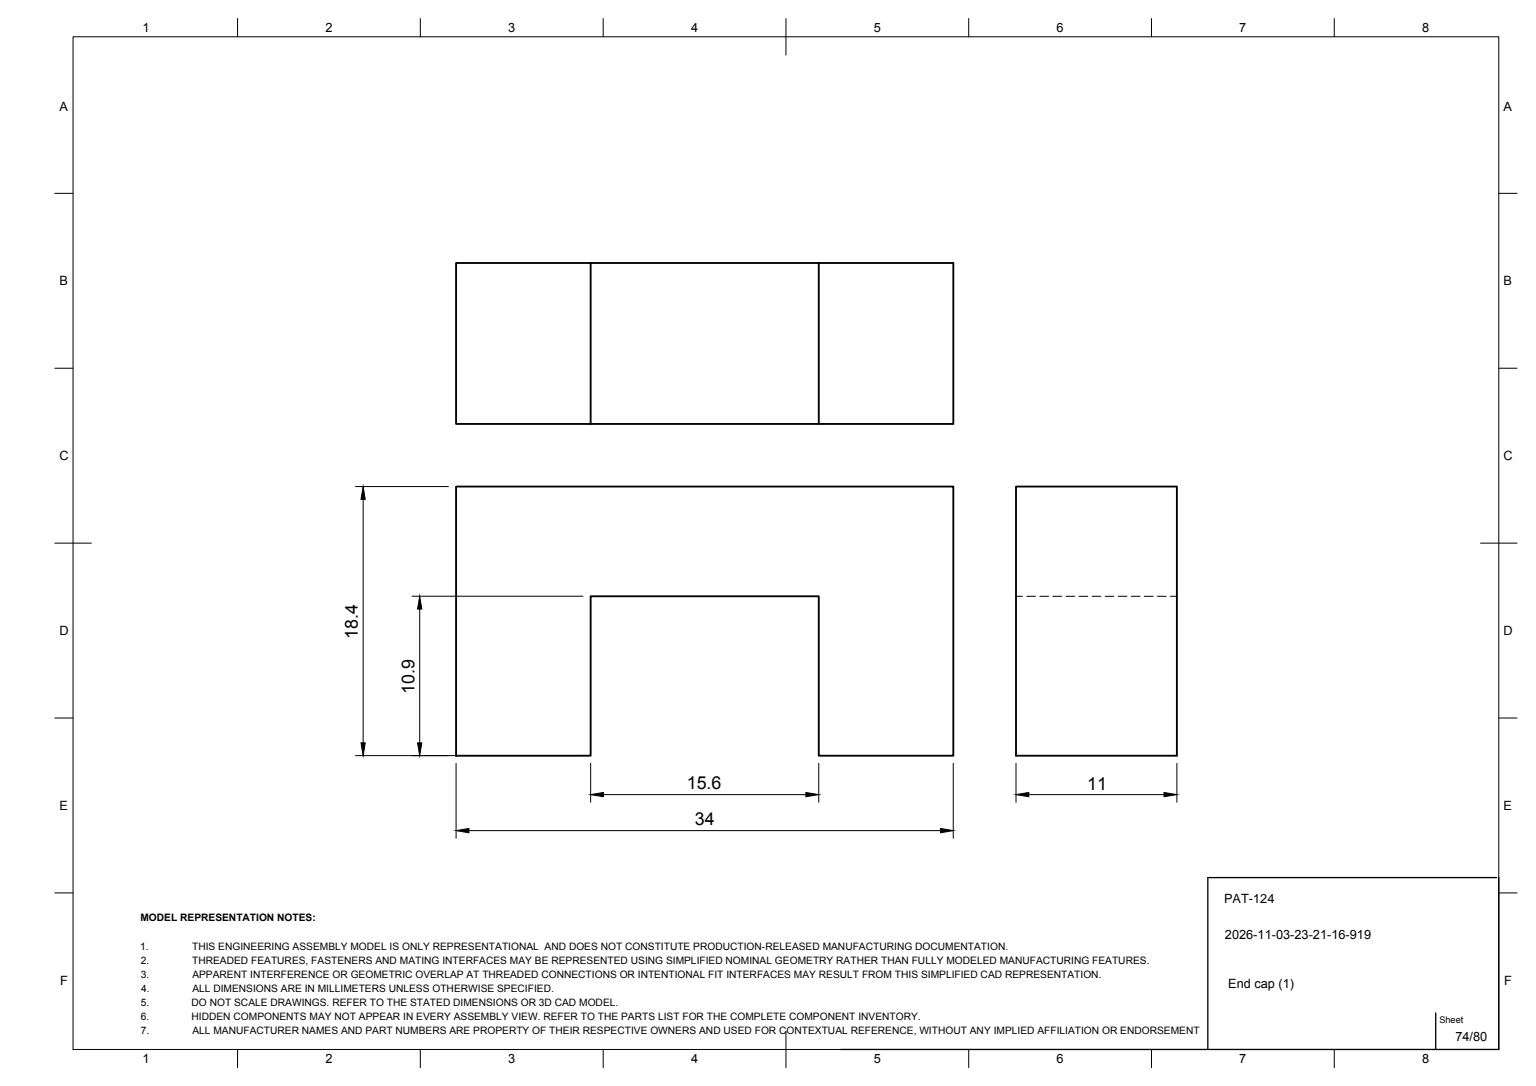
ISO-10303-21;
HEADER;
/* Generated by software containing ST-Developer
 * from STEP Tools, Inc. (www.steptools.com) 
 */

FILE_DESCRIPTION(
/* description */ ('XY cross-slide table'),
/* implementation_level */ '2;1');

FILE_NAME(
/* name */ 'End cap (1).step',
/* time_stamp */ '2026-10-28T03:22:46-07:00',
/* author */ (''),
/* organization */ (''),
/* preprocessor_version */ 'ST-DEVELOPER v20.2',
/* originating_system */ 'Autodesk Translation Framework v15.17.0.0',
/* authorisation */ '');

FILE_SCHEMA (('AUTOMOTIVE_DESIGN { 1 0 10303 214 3 1 1 }'));
ENDSEC;

DATA;
#10=MECHANICAL_DESIGN_GEOMETRIC_PRESENTATION_REPRESENTATION('',(#1767),#62984);
#1571=SHAPE_REPRESENTATION_RELATIONSHIP('SRR','None',#63430,#1654);
#1654=ADVANCED_BREP_SHAPE_REPRESENTATION('',(#1875),#62967);
#1767=STYLED_ITEM('',(#63926),#1875);
#1875=MANIFOLD_SOLID_BREP('Body1',#23066);
#2759=PLANE('',#25957);
#2760=PLANE('',#25958);
#2761=PLANE('',#25959);
#2762=PLANE('',#25960);
#2763=PLANE('',#25961);
#2764=PLANE('',#25962);
#2765=PLANE('',#25963);
#2766=PLANE('',#25964);
#2767=PLANE('',#25965);
#2768=PLANE('',#25966);
#3867=FACE_OUTER_BOUND('',#5551,.T.);
#3868=FACE_OUTER_BOUND('',#5552,.T.);
#3869=FACE_OUTER_BOUND('',#5553,.T.);
#3870=FACE_OUTER_BOUND('',#5554,.T.);
#3871=FACE_OUTER_BOUND('',#5555,.T.);
#3872=FACE_OUTER_BOUND('',#5556,.T.);
#3873=FACE_OUTER_BOUND('',#5557,.T.);
#3874=FACE_OUTER_BOUND('',#5558,.T.);
#3875=FACE_OUTER_BOUND('',#5559,.T.);
#3876=FACE_OUTER_BOUND('',#5560,.T.);
#5551=EDGE_LOOP('',(#19482,#19483,#19484,#19485));
#5552=EDGE_LOOP('',(#19486,#19487,#19488,#19489));
#5553=EDGE_LOOP('',(#19490,#19491,#19492,#19493));
#5554=EDGE_LOOP('',(#19494,#19495,#19496,#19497));
#5555=EDGE_LOOP('',(#19498,#19499,#19500,#19501));
#5556=EDGE_LOOP('',(#19502,#19503,#19504,#19505));
#5557=EDGE_LOOP('',(#19506,#19507,#19508,#19509));
#5558=EDGE_LOOP('',(#19510,#19511,#19512,#19513));
#5559=EDGE_LOOP('',(#19514,#19515,#19516,#19517,#19518,#19519,#19520,#19521));
#5560=EDGE_LOOP('',(#19522,#19523,#19524,#19525,#19526,#19527,#19528,#19529));
#7028=LINE('',#50118,#8515);
#7029=LINE('',#50120,#8516);
#7030=LINE('',#50122,#8517);
#7031=LINE('',#50123,#8518);
#7032=LINE('',#50126,#8519);
#7033=LINE('',#50128,#8520);
#7034=LINE('',#50129,#8521);
#7035=LINE('',#50132,#8522);
#7036=LINE('',#50134,#8523);
#7037=LINE('',#50135,#8524);
#7038=LINE('',#50138,#8525);
#7039=LINE('',#50140,#8526);
#7040=LINE('',#50141,#8527);
#7041=LINE('',#50144,#8528);
#7042=LINE('',#50146,#8529);
#7043=LINE('',#50147,#8530);
#7044=LINE('',#50150,#8531);
#7045=LINE('',#50152,#8532);
#7046=LINE('',#50153,#8533);
#7047=LINE('',#50156,#8534);
#7048=LINE('',#50158,#8535);
#7049=LINE('',#50159,#8536);
#7050=LINE('',#50161,#8537);
#7051=LINE('',#50162,#8538);
#8515=VECTOR('',#31499,1.);
#8516=VECTOR('',#31500,1.);
#8517=VECTOR('',#31501,1.);
#8518=VECTOR('',#31502,1.);
#8519=VECTOR('',#31505,1.);
#8520=VECTOR('',#31506,1.);
#8521=VECTOR('',#31507,1.);
#8522=VECTOR('',#31510,1.);
#8523=VECTOR('',#31511,1.);
#8524=VECTOR('',#31512,1.);
#8525=VECTOR('',#31515,1.);
#8526=VECTOR('',#31516,1.);
#8527=VECTOR('',#31517,1.);
#8528=VECTOR('',#31520,1.);
#8529=VECTOR('',#31521,1.);
#8530=VECTOR('',#31522,1.);
#8531=VECTOR('',#31525,1.);
#8532=VECTOR('',#31526,1.);
#8533=VECTOR('',#31527,1.);
#8534=VECTOR('',#31530,1.);
#8535=VECTOR('',#31531,1.);
#8536=VECTOR('',#31532,1.);
#8537=VECTOR('',#31535,1.);
#8538=VECTOR('',#31536,1.);
#11322=VERTEX_POINT('',#50116);
#11323=VERTEX_POINT('',#50117);
#11324=VERTEX_POINT('',#50119);
#11325=VERTEX_POINT('',#50121);
#11326=VERTEX_POINT('',#50125);
#11327=VERTEX_POINT('',#50127);
#11328=VERTEX_POINT('',#50131);
#11329=VERTEX_POINT('',#50133);
#11330=VERTEX_POINT('',#50137);
#11331=VERTEX_POINT('',#50139);
#11332=VERTEX_POINT('',#50143);
#11333=VERTEX_POINT('',#50145);
#11334=VERTEX_POINT('',#50149);
#11335=VERTEX_POINT('',#50151);
#11336=VERTEX_POINT('',#50155);
#11337=VERTEX_POINT('',#50157);
#14125=EDGE_CURVE('',#11322,#11323,#7028,.T.);
#14126=EDGE_CURVE('',#11322,#11324,#7029,.T.);
#14127=EDGE_CURVE('',#11325,#11324,#7030,.T.);
#14128=EDGE_CURVE('',#11323,#11325,#7031,.T.);
#14129=EDGE_CURVE('',#11323,#11326,#7032,.T.);
#14130=EDGE_CURVE('',#11327,#11325,#7033,.T.);
#14131=EDGE_CURVE('',#11326,#11327,#7034,.T.);
#14132=EDGE_CURVE('',#11326,#11328,#7035,.T.);
#14133=EDGE_CURVE('',#11329,#11327,#7036,.T.);
#14134=EDGE_CURVE('',#11328,#11329,#7037,.T.);
#14135=EDGE_CURVE('',#11328,#11330,#7038,.T.);
#14136=EDGE_CURVE('',#11331,#11329,#7039,.T.);
#14137=EDGE_CURVE('',#11330,#11331,#7040,.T.);
#14138=EDGE_CURVE('',#11330,#11332,#7041,.T.);
#14139=EDGE_CURVE('',#11333,#11331,#7042,.T.);
#14140=EDGE_CURVE('',#11332,#11333,#7043,.T.);
#14141=EDGE_CURVE('',#11332,#11334,#7044,.T.);
#14142=EDGE_CURVE('',#11335,#11333,#7045,.T.);
#14143=EDGE_CURVE('',#11334,#11335,#7046,.T.);
#14144=EDGE_CURVE('',#11334,#11336,#7047,.T.);
#14145=EDGE_CURVE('',#11337,#11335,#7048,.T.);
#14146=EDGE_CURVE('',#11336,#11337,#7049,.T.);
#14147=EDGE_CURVE('',#11336,#11322,#7050,.T.);
#14148=EDGE_CURVE('',#11324,#11337,#7051,.T.);
#19482=ORIENTED_EDGE('',*,*,#14125,.F.);
#19483=ORIENTED_EDGE('',*,*,#14126,.T.);
#19484=ORIENTED_EDGE('',*,*,#14127,.F.);
#19485=ORIENTED_EDGE('',*,*,#14128,.F.);
#19486=ORIENTED_EDGE('',*,*,#14129,.F.);
#19487=ORIENTED_EDGE('',*,*,#14128,.T.);
#19488=ORIENTED_EDGE('',*,*,#14130,.F.);
#19489=ORIENTED_EDGE('',*,*,#14131,.F.);
#19490=ORIENTED_EDGE('',*,*,#14132,.F.);
#19491=ORIENTED_EDGE('',*,*,#14131,.T.);
#19492=ORIENTED_EDGE('',*,*,#14133,.F.);
#19493=ORIENTED_EDGE('',*,*,#14134,.F.);
#19494=ORIENTED_EDGE('',*,*,#14135,.F.);
#19495=ORIENTED_EDGE('',*,*,#14134,.T.);
#19496=ORIENTED_EDGE('',*,*,#14136,.F.);
#19497=ORIENTED_EDGE('',*,*,#14137,.F.);
#19498=ORIENTED_EDGE('',*,*,#14138,.F.);
#19499=ORIENTED_EDGE('',*,*,#14137,.T.);
#19500=ORIENTED_EDGE('',*,*,#14139,.F.);
#19501=ORIENTED_EDGE('',*,*,#14140,.F.);
#19502=ORIENTED_EDGE('',*,*,#14141,.F.);
#19503=ORIENTED_EDGE('',*,*,#14140,.T.);
#19504=ORIENTED_EDGE('',*,*,#14142,.F.);
#19505=ORIENTED_EDGE('',*,*,#14143,.F.);
#19506=ORIENTED_EDGE('',*,*,#14144,.F.);
#19507=ORIENTED_EDGE('',*,*,#14143,.T.);
#19508=ORIENTED_EDGE('',*,*,#14145,.F.);
#19509=ORIENTED_EDGE('',*,*,#14146,.F.);
#19510=ORIENTED_EDGE('',*,*,#14147,.F.);
#19511=ORIENTED_EDGE('',*,*,#14146,.T.);
#19512=ORIENTED_EDGE('',*,*,#14148,.F.);
#19513=ORIENTED_EDGE('',*,*,#14126,.F.);
#19514=ORIENTED_EDGE('',*,*,#14147,.T.);
#19515=ORIENTED_EDGE('',*,*,#14125,.T.);
#19516=ORIENTED_EDGE('',*,*,#14129,.T.);
#19517=ORIENTED_EDGE('',*,*,#14132,.T.);
#19518=ORIENTED_EDGE('',*,*,#14135,.T.);
#19519=ORIENTED_EDGE('',*,*,#14138,.T.);
#19520=ORIENTED_EDGE('',*,*,#14141,.T.);
#19521=ORIENTED_EDGE('',*,*,#14144,.T.);
#19522=ORIENTED_EDGE('',*,*,#14148,.T.);
#19523=ORIENTED_EDGE('',*,*,#14145,.T.);
#19524=ORIENTED_EDGE('',*,*,#14142,.T.);
#19525=ORIENTED_EDGE('',*,*,#14139,.T.);
#19526=ORIENTED_EDGE('',*,*,#14136,.T.);
#19527=ORIENTED_EDGE('',*,*,#14133,.T.);
#19528=ORIENTED_EDGE('',*,*,#14130,.T.);
#19529=ORIENTED_EDGE('',*,*,#14127,.T.);
#22648=ADVANCED_FACE('',(#3867),#2759,.T.);
#22649=ADVANCED_FACE('',(#3868),#2760,.T.);
#22650=ADVANCED_FACE('',(#3869),#2761,.T.);
#22651=ADVANCED_FACE('',(#3870),#2762,.T.);
#22652=ADVANCED_FACE('',(#3871),#2763,.T.);
#22653=ADVANCED_FACE('',(#3872),#2764,.T.);
#22654=ADVANCED_FACE('',(#3873),#2765,.T.);
#22655=ADVANCED_FACE('',(#3874),#2766,.T.);
#22656=ADVANCED_FACE('',(#3875),#2767,.T.);
#22657=ADVANCED_FACE('',(#3876),#2768,.T.);
#23066=CLOSED_SHELL('',(#22648,#22649,#22650,#22651,#22652,#22653,#22654,
#22655,#22656,#22657));
#25956=AXIS2_PLACEMENT_3D('',#50114,#31495,#31496);
#25957=AXIS2_PLACEMENT_3D('',#50115,#31497,#31498);
#25958=AXIS2_PLACEMENT_3D('',#50124,#31503,#31504);
#25959=AXIS2_PLACEMENT_3D('',#50130,#31508,#31509);
#25960=AXIS2_PLACEMENT_3D('',#50136,#31513,#31514);
#25961=AXIS2_PLACEMENT_3D('',#50142,#31518,#31519);
#25962=AXIS2_PLACEMENT_3D('',#50148,#31523,#31524);
#25963=AXIS2_PLACEMENT_3D('',#50154,#31528,#31529);
#25964=AXIS2_PLACEMENT_3D('',#50160,#31533,#31534);
#25965=AXIS2_PLACEMENT_3D('',#50163,#31537,#31538);
#25966=AXIS2_PLACEMENT_3D('',#50164,#31539,#31540);
#31495=DIRECTION('axis',(0.,0.,1.));
#31496=DIRECTION('refdir',(1.,0.,0.));
#31497=DIRECTION('center_axis',(0.,0.,-1.));
#31498=DIRECTION('ref_axis',(0.,-1.,0.));
#31499=DIRECTION('',(0.,1.,0.));
#31500=DIRECTION('',(-1.,0.,0.));
#31501=DIRECTION('',(0.,-1.,0.));
#31502=DIRECTION('',(-1.,0.,0.));
#31503=DIRECTION('center_axis',(0.,1.,0.));
#31504=DIRECTION('ref_axis',(0.,0.,-1.));
#31505=DIRECTION('',(0.,0.,1.));
#31506=DIRECTION('',(0.,0.,-1.));
#31507=DIRECTION('',(-1.,0.,0.));
#31508=DIRECTION('center_axis',(0.,0.,-1.));
#31509=DIRECTION('ref_axis',(0.,-1.,0.));
#31510=DIRECTION('',(0.,1.,0.));
#31511=DIRECTION('',(0.,-1.,0.));
#31512=DIRECTION('',(-1.,0.,0.));
#31513=DIRECTION('center_axis',(0.,-1.,0.));
#31514=DIRECTION('ref_axis',(0.,0.,1.));
#31515=DIRECTION('',(0.,0.,-1.));
#31516=DIRECTION('',(0.,0.,1.));
#31517=DIRECTION('',(-1.,0.,0.));
#31518=DIRECTION('center_axis',(0.,0.,-1.));
#31519=DIRECTION('ref_axis',(0.,-1.,0.));
#31520=DIRECTION('',(0.,1.,0.));
#31521=DIRECTION('',(0.,-1.,0.));
#31522=DIRECTION('',(-1.,0.,0.));
#31523=DIRECTION('center_axis',(0.,1.,0.));
#31524=DIRECTION('ref_axis',(0.,0.,-1.));
#31525=DIRECTION('',(0.,0.,1.));
#31526=DIRECTION('',(0.,0.,-1.));
#31527=DIRECTION('',(-1.,0.,0.));
#31528=DIRECTION('center_axis',(0.,0.,1.));
#31529=DIRECTION('ref_axis',(0.,1.,0.));
#31530=DIRECTION('',(0.,-1.,0.));
#31531=DIRECTION('',(0.,1.,0.));
#31532=DIRECTION('',(-1.,0.,0.));
#31533=DIRECTION('center_axis',(0.,-1.,0.));
#31534=DIRECTION('ref_axis',(0.,0.,1.));
#31535=DIRECTION('',(0.,0.,-1.));
#31536=DIRECTION('',(0.,0.,1.));
#31537=DIRECTION('center_axis',(1.,0.,0.));
#31538=DIRECTION('ref_axis',(0.,0.,-1.));
#31539=DIRECTION('center_axis',(-1.,0.,0.));
#31540=DIRECTION('ref_axis',(0.,0.,1.));
#50114=CARTESIAN_POINT('',(0.,0.,0.));
#50115=CARTESIAN_POINT('Origin',(-1.97,-0.78,0.46));
#50116=CARTESIAN_POINT('',(-1.97,-1.7,0.46));
#50117=CARTESIAN_POINT('',(-1.97,-0.78,0.46));
#50118=CARTESIAN_POINT('',(-1.97,-1.7,0.46));
#50119=CARTESIAN_POINT('',(-3.07,-1.7,0.46));
#50120=CARTESIAN_POINT('',(-1.97,-1.7,0.46));
#50121=CARTESIAN_POINT('',(-3.07,-0.78,0.46));
#50122=CARTESIAN_POINT('',(-3.07,-1.7,0.46));
#50123=CARTESIAN_POINT('',(-1.97,-0.78,0.46));
#50124=CARTESIAN_POINT('Origin',(-1.97,-0.78,1.55));
#50125=CARTESIAN_POINT('',(-1.97,-0.78,1.55));
#50126=CARTESIAN_POINT('',(-1.97,-0.78,0.46));
#50127=CARTESIAN_POINT('',(-3.07,-0.78,1.55));
#50128=CARTESIAN_POINT('',(-3.07,-0.78,0.46));
#50129=CARTESIAN_POINT('',(-1.97,-0.78,1.55));
#50130=CARTESIAN_POINT('Origin',(-1.97,0.78,1.55));
#50131=CARTESIAN_POINT('',(-1.97,0.78,1.55));
#50132=CARTESIAN_POINT('',(-1.97,-0.78,1.55));
#50133=CARTESIAN_POINT('',(-3.07,0.78,1.55));
#50134=CARTESIAN_POINT('',(-3.07,-0.78,1.55));
#50135=CARTESIAN_POINT('',(-1.97,0.78,1.55));
#50136=CARTESIAN_POINT('Origin',(-1.97,0.78,0.46));
#50137=CARTESIAN_POINT('',(-1.97,0.78,0.46));
#50138=CARTESIAN_POINT('',(-1.97,0.78,1.55));
#50139=CARTESIAN_POINT('',(-3.07,0.78,0.46));
#50140=CARTESIAN_POINT('',(-3.07,0.78,1.55));
#50141=CARTESIAN_POINT('',(-1.97,0.78,0.46));
#50142=CARTESIAN_POINT('Origin',(-1.97,1.7,0.46));
#50143=CARTESIAN_POINT('',(-1.97,1.7,0.46));
#50144=CARTESIAN_POINT('',(-1.97,0.78,0.46));
#50145=CARTESIAN_POINT('',(-3.07,1.7,0.46));
#50146=CARTESIAN_POINT('',(-3.07,0.78,0.46));
#50147=CARTESIAN_POINT('',(-1.97,1.7,0.46));
#50148=CARTESIAN_POINT('Origin',(-1.97,1.7,2.3));
#50149=CARTESIAN_POINT('',(-1.97,1.7,2.3));
#50150=CARTESIAN_POINT('',(-1.97,1.7,0.46));
#50151=CARTESIAN_POINT('',(-3.07,1.7,2.3));
#50152=CARTESIAN_POINT('',(-3.07,1.7,0.46));
#50153=CARTESIAN_POINT('',(-1.97,1.7,2.3));
#50154=CARTESIAN_POINT('Origin',(-1.97,-1.7,2.3));
#50155=CARTESIAN_POINT('',(-1.97,-1.7,2.3));
#50156=CARTESIAN_POINT('',(-1.97,1.7,2.3));
#50157=CARTESIAN_POINT('',(-3.07,-1.7,2.3));
#50158=CARTESIAN_POINT('',(-3.07,1.7,2.3));
#50159=CARTESIAN_POINT('',(-1.97,-1.7,2.3));
#50160=CARTESIAN_POINT('Origin',(-1.97,-1.7,0.46));
#50161=CARTESIAN_POINT('',(-1.97,-1.7,2.3));
#50162=CARTESIAN_POINT('',(-3.07,-1.7,2.3));
#50163=CARTESIAN_POINT('Origin',(-1.97,0.,1.38));
#50164=CARTESIAN_POINT('Origin',(-3.07,0.,1.38));
#62868=UNCERTAINTY_MEASURE_WITH_UNIT(LENGTH_MEASURE(0.001),#62985,
'DISTANCE_ACCURACY_VALUE',
'Maximum model space distance between geometric entities at asserted c
onnectivities');
#62885=UNCERTAINTY_MEASURE_WITH_UNIT(LENGTH_MEASURE(0.001),#62985,
'DISTANCE_ACCURACY_VALUE',
'Maximum model space distance between geometric entities at asserted c
onnectivities');
#62967=(
GEOMETRIC_REPRESENTATION_CONTEXT(3)
GLOBAL_UNCERTAINTY_ASSIGNED_CONTEXT((#62868))
GLOBAL_UNIT_ASSIGNED_CONTEXT((#62985,#62987,#62988))
REPRESENTATION_CONTEXT('','3D')
);
#62984=(
GEOMETRIC_REPRESENTATION_CONTEXT(3)
GLOBAL_UNCERTAINTY_ASSIGNED_CONTEXT((#62885))
GLOBAL_UNIT_ASSIGNED_CONTEXT((#62985,#62987,#62988))
REPRESENTATION_CONTEXT('','3D')
);
#62985=(
LENGTH_UNIT()
NAMED_UNIT(*)
SI_UNIT(.CENTI.,.METRE.)
);
#62987=(
NAMED_UNIT(*)
PLANE_ANGLE_UNIT()
SI_UNIT($,.RADIAN.)
);
#62988=(
NAMED_UNIT(*)
SI_UNIT($,.STERADIAN.)
SOLID_ANGLE_UNIT()
);
#63070=SHAPE_DEFINITION_REPRESENTATION(#63258,#63430);
#63258=PRODUCT_DEFINITION_SHAPE('',$,#63529);
#63430=SHAPE_REPRESENTATION('',(#25956),#62967);
#63447=PRODUCT_DEFINITION_CONTEXT('part definition',#63743,'design');
#63529=PRODUCT_DEFINITION('End cap (1)','End cap (1)',#63627,#63447);
#63627=PRODUCT_DEFINITION_FORMATION('',$,#63826);
#63743=APPLICATION_CONTEXT(
'Core Data for Automotive Mechanical Design Process');
#63744=PRODUCT_CONTEXT('part definition',#63743,'mechanical');
#63826=PRODUCT('End cap (1)','End cap (1)','End cap (1)',(#63744));
#63920=COLOUR_RGB('Off White',0.89,0.88,0.83);
#63921=FILL_AREA_STYLE_COLOUR('',#63920);
#63922=FILL_AREA_STYLE('',(#63921));
#63923=SURFACE_STYLE_FILL_AREA(#63922);
#63924=SURFACE_SIDE_STYLE('',(#63923));
#63925=SURFACE_STYLE_USAGE(.BOTH.,#63924);
#63926=PRESENTATION_STYLE_ASSIGNMENT((#63925));
ENDSEC;
END-ISO-10303-21;
